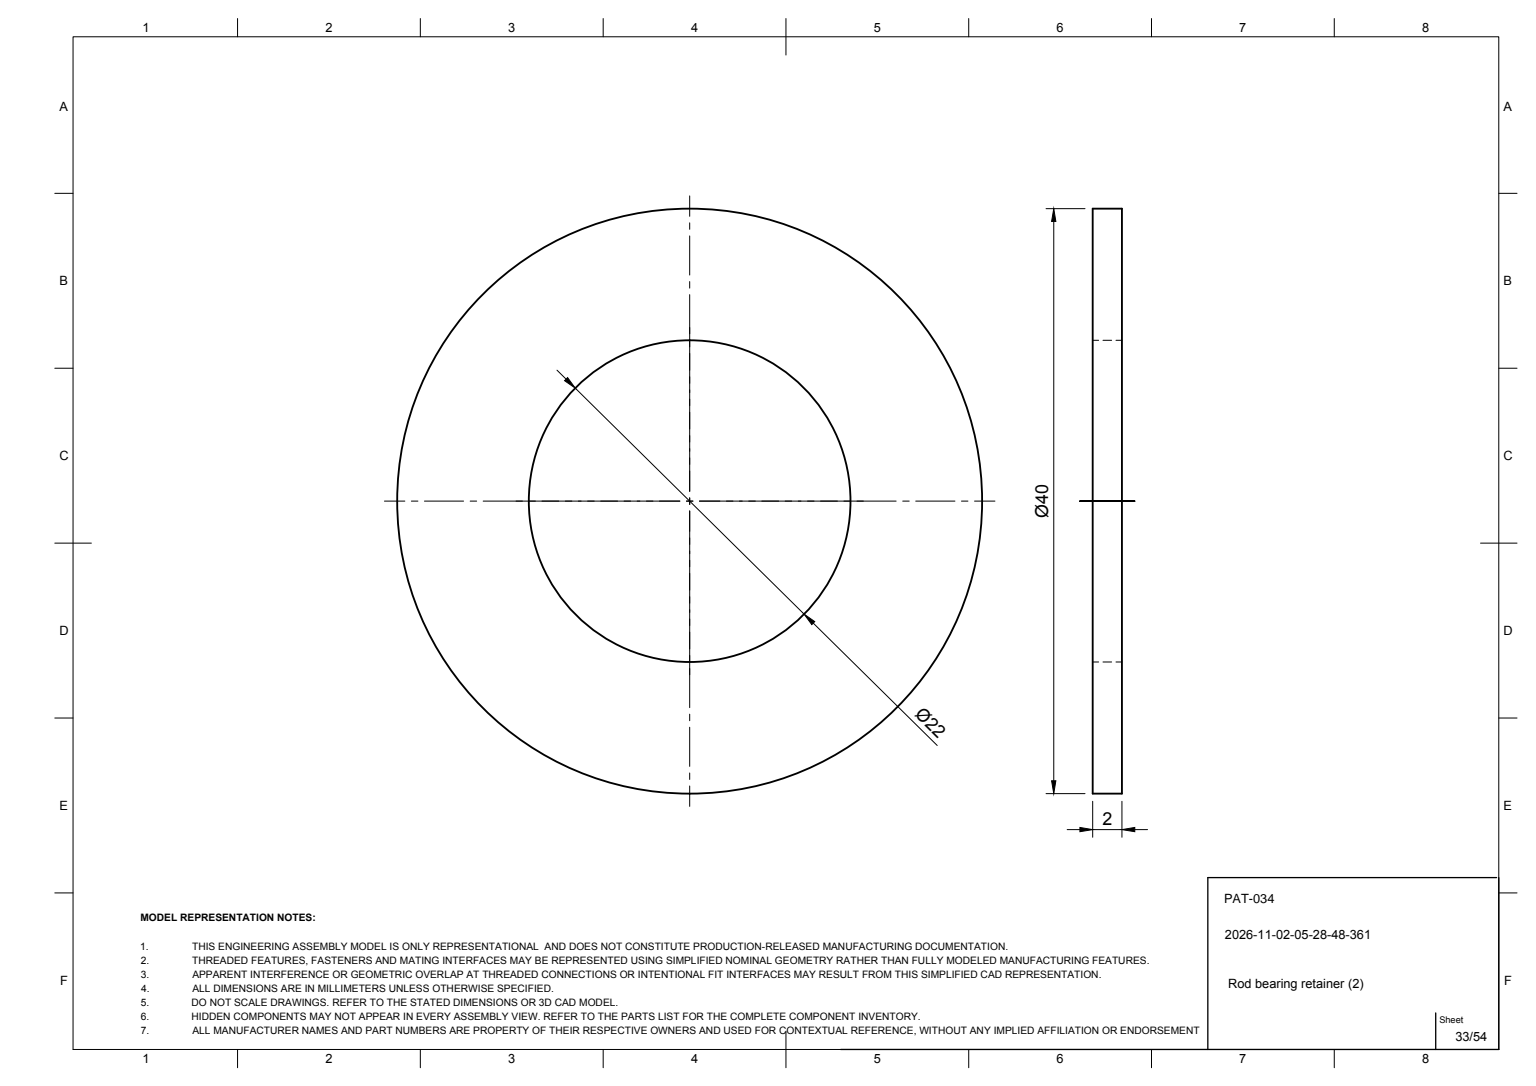
ISO-10303-21;
HEADER;
/* Generated by software containing ST-Developer
 * from STEP Tools, Inc. (www.steptools.com) 
 */

FILE_DESCRIPTION(
/* description */ ('Fatigue rig crank-slider'),
/* implementation_level */ '2;1');

FILE_NAME(
/* name */ 'Rod bearing retainer (2).step',
/* time_stamp */ '2026-10-28T03:24:50-07:00',
/* author */ (''),
/* organization */ (''),
/* preprocessor_version */ 'ST-DEVELOPER v20.2',
/* originating_system */ 'Autodesk Translation Framework v15.17.0.0',
/* authorisation */ '');

FILE_SCHEMA (('AUTOMOTIVE_DESIGN { 1 0 10303 214 3 1 1 }'));
ENDSEC;

DATA;
#10=MECHANICAL_DESIGN_GEOMETRIC_PRESENTATION_REPRESENTATION('',(#618),#16911);
#517=SHAPE_REPRESENTATION_RELATIONSHIP('SRR','None',#17159,#567);
#567=ADVANCED_BREP_SHAPE_REPRESENTATION('',(#675),#16888);
#618=STYLED_ITEM('',(#17487),#675);
#675=MANIFOLD_SOLID_BREP('Body1',#8911);
#850=FACE_BOUND('',#2210,.T.);
#851=FACE_BOUND('',#2212,.T.);
#1090=PLANE('',#10095);
#1091=PLANE('',#10096);
#1534=FACE_OUTER_BOUND('',#2207,.T.);
#1535=FACE_OUTER_BOUND('',#2208,.T.);
#1536=FACE_OUTER_BOUND('',#2209,.T.);
#1537=FACE_OUTER_BOUND('',#2211,.T.);
#2207=EDGE_LOOP('',(#7316,#7317,#7318,#7319));
#2208=EDGE_LOOP('',(#7320,#7321,#7322,#7323));
#2209=EDGE_LOOP('',(#7324));
#2210=EDGE_LOOP('',(#7325));
#2211=EDGE_LOOP('',(#7326));
#2212=EDGE_LOOP('',(#7327));
#2843=LINE('',#15403,#3489);
#2844=LINE('',#15409,#3490);
#3489=VECTOR('',#12145,1.1);
#3490=VECTOR('',#12152,2.);
#3993=CIRCLE('',#10090,1.1);
#3994=CIRCLE('',#10091,1.1);
#3995=CIRCLE('',#10093,2.);
#3996=CIRCLE('',#10094,2.);
#4597=VERTEX_POINT('',#15400);
#4598=VERTEX_POINT('',#15402);
#4599=VERTEX_POINT('',#15406);
#4600=VERTEX_POINT('',#15408);
#5556=EDGE_CURVE('',#4597,#4597,#3993,.T.);
#5557=EDGE_CURVE('',#4597,#4598,#2843,.T.);
#5558=EDGE_CURVE('',#4598,#4598,#3994,.T.);
#5559=EDGE_CURVE('',#4599,#4599,#3995,.T.);
#5560=EDGE_CURVE('',#4599,#4600,#2844,.T.);
#5561=EDGE_CURVE('',#4600,#4600,#3996,.T.);
#7316=ORIENTED_EDGE('',*,*,#5556,.F.);
#7317=ORIENTED_EDGE('',*,*,#5557,.T.);
#7318=ORIENTED_EDGE('',*,*,#5558,.T.);
#7319=ORIENTED_EDGE('',*,*,#5557,.F.);
#7320=ORIENTED_EDGE('',*,*,#5559,.F.);
#7321=ORIENTED_EDGE('',*,*,#5560,.T.);
#7322=ORIENTED_EDGE('',*,*,#5561,.T.);
#7323=ORIENTED_EDGE('',*,*,#5560,.F.);
#7324=ORIENTED_EDGE('',*,*,#5559,.T.);
#7325=ORIENTED_EDGE('',*,*,#5556,.T.);
#7326=ORIENTED_EDGE('',*,*,#5561,.F.);
#7327=ORIENTED_EDGE('',*,*,#5558,.F.);
#8309=CYLINDRICAL_SURFACE('',#10089,1.1);
#8310=CYLINDRICAL_SURFACE('',#10092,2.);
#8672=ADVANCED_FACE('',(#1534),#8309,.F.);
#8673=ADVANCED_FACE('',(#1535),#8310,.T.);
#8674=ADVANCED_FACE('',(#1536,#850),#1090,.T.);
#8675=ADVANCED_FACE('',(#1537,#851),#1091,.F.);
#8911=CLOSED_SHELL('',(#8672,#8673,#8674,#8675));
#10088=AXIS2_PLACEMENT_3D('',#15398,#12139,#12140);
#10089=AXIS2_PLACEMENT_3D('',#15399,#12141,#12142);
#10090=AXIS2_PLACEMENT_3D('',#15401,#12143,#12144);
#10091=AXIS2_PLACEMENT_3D('',#15404,#12146,#12147);
#10092=AXIS2_PLACEMENT_3D('',#15405,#12148,#12149);
#10093=AXIS2_PLACEMENT_3D('',#15407,#12150,#12151);
#10094=AXIS2_PLACEMENT_3D('',#15410,#12153,#12154);
#10095=AXIS2_PLACEMENT_3D('',#15411,#12155,#12156);
#10096=AXIS2_PLACEMENT_3D('',#15412,#12157,#12158);
#12139=DIRECTION('axis',(0.,0.,1.));
#12140=DIRECTION('refdir',(1.,0.,0.));
#12141=DIRECTION('center_axis',(0.,1.,0.));
#12142=DIRECTION('ref_axis',(1.,0.,0.));
#12143=DIRECTION('center_axis',(0.,-1.,0.));
#12144=DIRECTION('ref_axis',(1.,0.,0.));
#12145=DIRECTION('',(0.,-1.,0.));
#12146=DIRECTION('center_axis',(0.,-1.,0.));
#12147=DIRECTION('ref_axis',(1.,0.,0.));
#12148=DIRECTION('center_axis',(0.,1.,0.));
#12149=DIRECTION('ref_axis',(1.,0.,0.));
#12150=DIRECTION('center_axis',(0.,1.,0.));
#12151=DIRECTION('ref_axis',(1.,0.,0.));
#12152=DIRECTION('',(0.,-1.,0.));
#12153=DIRECTION('center_axis',(0.,1.,0.));
#12154=DIRECTION('ref_axis',(1.,0.,0.));
#12155=DIRECTION('center_axis',(0.,1.,0.));
#12156=DIRECTION('ref_axis',(1.,0.,0.));
#12157=DIRECTION('center_axis',(0.,1.,0.));
#12158=DIRECTION('ref_axis',(1.,0.,0.));
#15398=CARTESIAN_POINT('',(0.,0.,0.));
#15399=CARTESIAN_POINT('Origin',(11.,3.3,12.));
#15400=CARTESIAN_POINT('',(9.9,3.5,12.));
#15401=CARTESIAN_POINT('Origin',(11.,3.5,12.));
#15402=CARTESIAN_POINT('',(9.9,3.3,12.));
#15403=CARTESIAN_POINT('',(9.9,3.3,12.));
#15404=CARTESIAN_POINT('Origin',(11.,3.3,12.));
#15405=CARTESIAN_POINT('Origin',(11.,3.3,12.));
#15406=CARTESIAN_POINT('',(9.,3.5,12.));
#15407=CARTESIAN_POINT('Origin',(11.,3.5,12.));
#15408=CARTESIAN_POINT('',(9.,3.3,12.));
#15409=CARTESIAN_POINT('',(9.,3.3,12.));
#15410=CARTESIAN_POINT('Origin',(11.,3.3,12.));
#15411=CARTESIAN_POINT('Origin',(11.,3.5,12.));
#15412=CARTESIAN_POINT('Origin',(11.,3.3,12.));
#16829=UNCERTAINTY_MEASURE_WITH_UNIT(LENGTH_MEASURE(0.001),#16912,
'DISTANCE_ACCURACY_VALUE',
'Maximum model space distance between geometric entities at asserted c
onnectivities');
#16852=UNCERTAINTY_MEASURE_WITH_UNIT(LENGTH_MEASURE(0.001),#16912,
'DISTANCE_ACCURACY_VALUE',
'Maximum model space distance between geometric entities at asserted c
onnectivities');
#16888=(
GEOMETRIC_REPRESENTATION_CONTEXT(3)
GLOBAL_UNCERTAINTY_ASSIGNED_CONTEXT((#16829))
GLOBAL_UNIT_ASSIGNED_CONTEXT((#16912,#16914,#16915))
REPRESENTATION_CONTEXT('','3D')
);
#16911=(
GEOMETRIC_REPRESENTATION_CONTEXT(3)
GLOBAL_UNCERTAINTY_ASSIGNED_CONTEXT((#16852))
GLOBAL_UNIT_ASSIGNED_CONTEXT((#16912,#16914,#16915))
REPRESENTATION_CONTEXT('','3D')
);
#16912=(
LENGTH_UNIT()
NAMED_UNIT(*)
SI_UNIT(.CENTI.,.METRE.)
);
#16914=(
NAMED_UNIT(*)
PLANE_ANGLE_UNIT()
SI_UNIT($,.RADIAN.)
);
#16915=(
NAMED_UNIT(*)
SI_UNIT($,.STERADIAN.)
SOLID_ANGLE_UNIT()
);
#16951=SHAPE_DEFINITION_REPRESENTATION(#17011,#17159);
#17011=PRODUCT_DEFINITION_SHAPE('',$,#17218);
#17159=SHAPE_REPRESENTATION('',(#10088),#16888);
#17182=PRODUCT_DEFINITION_CONTEXT('part definition',#17358,'design');
#17218=PRODUCT_DEFINITION('Rod bearing retainer (2)',
'Rod bearing retainer (2)',#17276,#17182);
#17276=PRODUCT_DEFINITION_FORMATION('',$,#17395);
#17358=APPLICATION_CONTEXT(
'Core Data for Automotive Mechanical Design Process');
#17359=PRODUCT_CONTEXT('part definition',#17358,'mechanical');
#17395=PRODUCT('Rod bearing retainer (2)','Rod bearing retainer (2)',
'Rod bearing retainer (2)',(#17359));
#17481=COLOUR_RGB('Grey',0.48,0.52,0.57);
#17482=FILL_AREA_STYLE_COLOUR('',#17481);
#17483=FILL_AREA_STYLE('',(#17482));
#17484=SURFACE_STYLE_FILL_AREA(#17483);
#17485=SURFACE_SIDE_STYLE('',(#17484));
#17486=SURFACE_STYLE_USAGE(.BOTH.,#17485);
#17487=PRESENTATION_STYLE_ASSIGNMENT((#17486));
ENDSEC;
END-ISO-10303-21;
